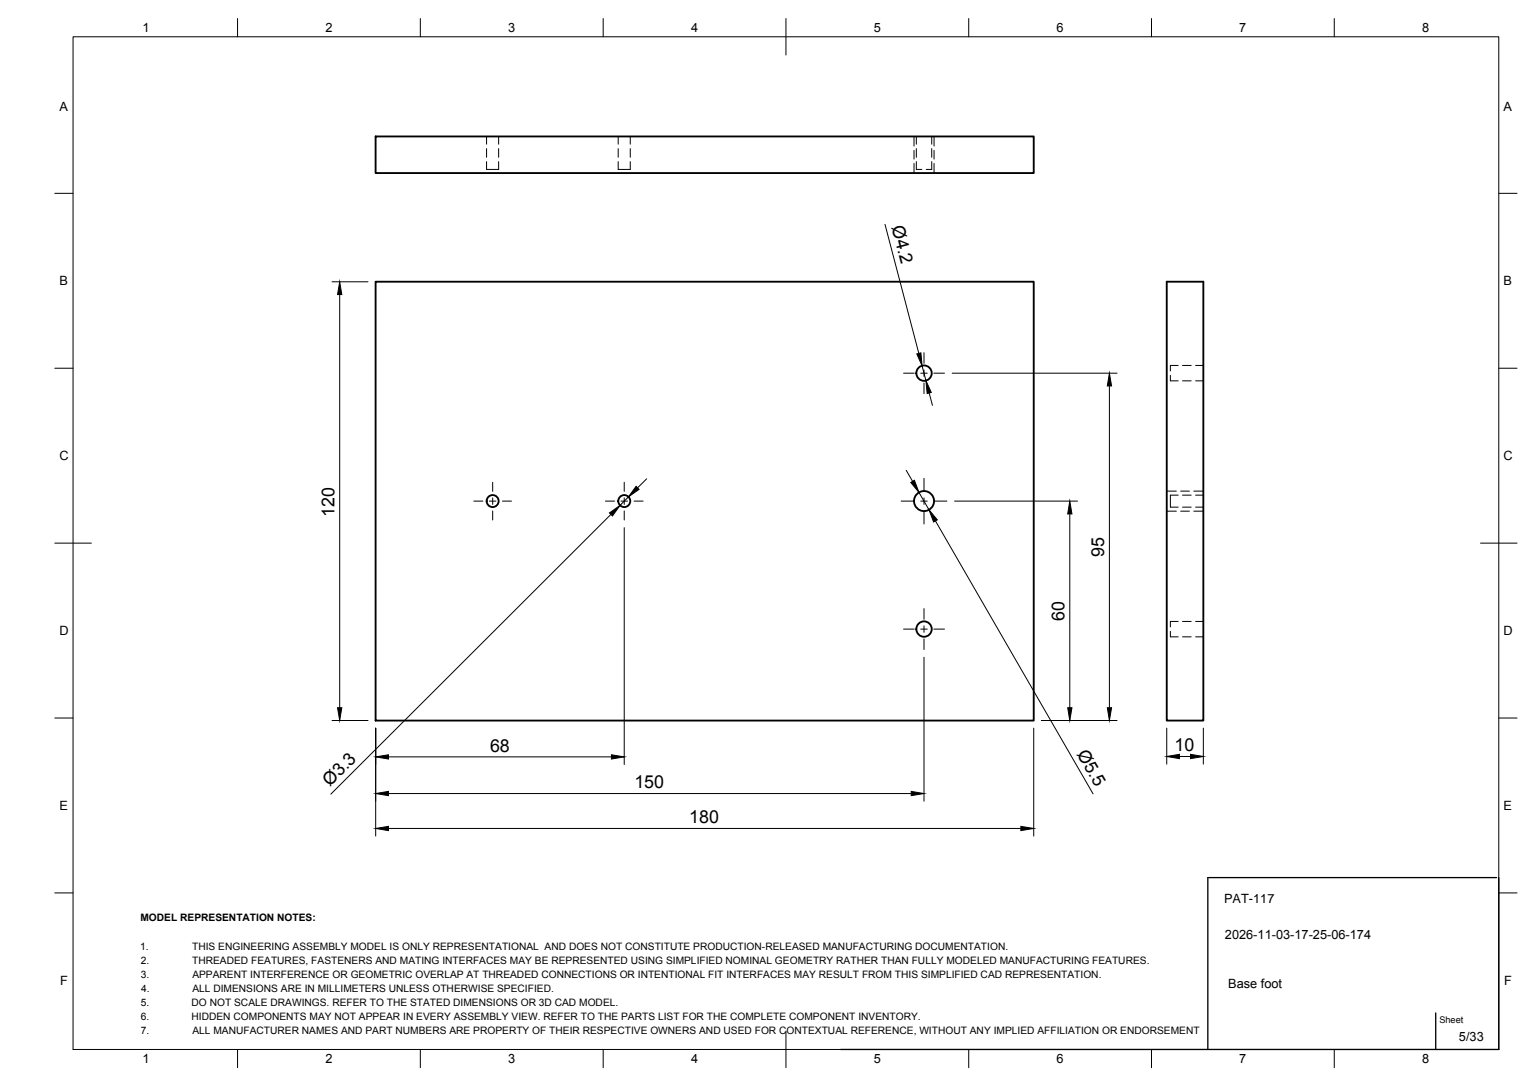
ISO-10303-21;
HEADER;
/* Generated by software containing ST-Developer
 * from STEP Tools, Inc. (www.steptools.com) 
 */

FILE_DESCRIPTION(
/* description */ ('Counterbalanced vertical column'),
/* implementation_level */ '2;1');

FILE_NAME(
/* name */ 'Base foot.step',
/* time_stamp */ '2026-10-29T16:47:22-07:00',
/* author */ (''),
/* organization */ (''),
/* preprocessor_version */ 'ST-DEVELOPER v20.2',
/* originating_system */ 'Autodesk Translation Framework v15.17.0.0',
/* authorisation */ '');

FILE_SCHEMA (('AUTOMOTIVE_DESIGN { 1 0 10303 214 3 1 1 }'));
ENDSEC;

DATA;
#10=MECHANICAL_DESIGN_GEOMETRIC_PRESENTATION_REPRESENTATION('',(#350),#15040);
#280=SHAPE_REPRESENTATION_RELATIONSHIP('SRR','None',#15184,#315);
#315=ADVANCED_BREP_SHAPE_REPRESENTATION('',(#385),#15003);
#350=STYLED_ITEM('',(#15436),#385);
#385=MANIFOLD_SOLID_BREP('Body1',#7073);
#416=FACE_BOUND('',#1245,.T.);
#417=FACE_BOUND('',#1246,.T.);
#418=FACE_BOUND('',#1247,.T.);
#419=FACE_BOUND('',#1248,.T.);
#420=FACE_BOUND('',#1249,.T.);
#421=FACE_BOUND('',#1251,.T.);
#531=PLANE('',#7504);
#532=PLANE('',#7508);
#533=PLANE('',#7512);
#534=PLANE('',#7516);
#535=PLANE('',#7520);
#536=PLANE('',#7521);
#537=PLANE('',#7522);
#538=PLANE('',#7523);
#539=PLANE('',#7524);
#540=PLANE('',#7525);
#826=FACE_OUTER_BOUND('',#1231,.T.);
#827=FACE_OUTER_BOUND('',#1232,.T.);
#828=FACE_OUTER_BOUND('',#1233,.T.);
#829=FACE_OUTER_BOUND('',#1234,.T.);
#830=FACE_OUTER_BOUND('',#1235,.T.);
#831=FACE_OUTER_BOUND('',#1236,.T.);
#832=FACE_OUTER_BOUND('',#1237,.T.);
#833=FACE_OUTER_BOUND('',#1238,.T.);
#834=FACE_OUTER_BOUND('',#1239,.T.);
#835=FACE_OUTER_BOUND('',#1240,.T.);
#836=FACE_OUTER_BOUND('',#1241,.T.);
#837=FACE_OUTER_BOUND('',#1242,.T.);
#838=FACE_OUTER_BOUND('',#1243,.T.);
#839=FACE_OUTER_BOUND('',#1244,.T.);
#840=FACE_OUTER_BOUND('',#1250,.T.);
#1231=EDGE_LOOP('',(#4788,#4789,#4790,#4791));
#1232=EDGE_LOOP('',(#4792));
#1233=EDGE_LOOP('',(#4793,#4794,#4795,#4796));
#1234=EDGE_LOOP('',(#4797));
#1235=EDGE_LOOP('',(#4798,#4799,#4800,#4801));
#1236=EDGE_LOOP('',(#4802));
#1237=EDGE_LOOP('',(#4803,#4804,#4805,#4806));
#1238=EDGE_LOOP('',(#4807));
#1239=EDGE_LOOP('',(#4808,#4809,#4810,#4811));
#1240=EDGE_LOOP('',(#4812,#4813,#4814,#4815));
#1241=EDGE_LOOP('',(#4816,#4817,#4818,#4819));
#1242=EDGE_LOOP('',(#4820,#4821,#4822,#4823));
#1243=EDGE_LOOP('',(#4824,#4825,#4826,#4827));
#1244=EDGE_LOOP('',(#4828,#4829,#4830,#4831));
#1245=EDGE_LOOP('',(#4832));
#1246=EDGE_LOOP('',(#4833));
#1247=EDGE_LOOP('',(#4834));
#1248=EDGE_LOOP('',(#4835));
#1249=EDGE_LOOP('',(#4836));
#1250=EDGE_LOOP('',(#4837,#4838,#4839,#4840));
#1251=EDGE_LOOP('',(#4841));
#1751=LINE('',#10345,#2422);
#1752=LINE('',#10352,#2423);
#1753=LINE('',#10359,#2424);
#1754=LINE('',#10366,#2425);
#1755=LINE('',#10373,#2426);
#1756=LINE('',#10378,#2427);
#1757=LINE('',#10380,#2428);
#1758=LINE('',#10382,#2429);
#1759=LINE('',#10383,#2430);
#1760=LINE('',#10386,#2431);
#1761=LINE('',#10388,#2432);
#1762=LINE('',#10389,#2433);
#1763=LINE('',#10392,#2434);
#1764=LINE('',#10394,#2435);
#1765=LINE('',#10395,#2436);
#1766=LINE('',#10397,#2437);
#1767=LINE('',#10398,#2438);
#2422=VECTOR('',#8231,0.21);
#2423=VECTOR('',#8240,0.21);
#2424=VECTOR('',#8249,0.165);
#2425=VECTOR('',#8258,0.164999999999999);
#2426=VECTOR('',#8267,0.275);
#2427=VECTOR('',#8272,1.);
#2428=VECTOR('',#8273,1.);
#2429=VECTOR('',#8274,1.);
#2430=VECTOR('',#8275,1.);
#2431=VECTOR('',#8278,1.);
#2432=VECTOR('',#8279,1.);
#2433=VECTOR('',#8280,1.);
#2434=VECTOR('',#8283,1.);
#2435=VECTOR('',#8284,1.);
#2436=VECTOR('',#8285,1.);
#2437=VECTOR('',#8288,1.);
#2438=VECTOR('',#8289,1.);
#3093=CIRCLE('',#7502,0.21);
#3094=CIRCLE('',#7503,0.21);
#3095=CIRCLE('',#7506,0.21);
#3096=CIRCLE('',#7507,0.21);
#3097=CIRCLE('',#7510,0.165);
#3098=CIRCLE('',#7511,0.165);
#3099=CIRCLE('',#7514,0.164999999999999);
#3100=CIRCLE('',#7515,0.164999999999999);
#3101=CIRCLE('',#7518,0.275);
#3102=CIRCLE('',#7519,0.275);
#3306=VERTEX_POINT('',#10342);
#3307=VERTEX_POINT('',#10344);
#3308=VERTEX_POINT('',#10349);
#3309=VERTEX_POINT('',#10351);
#3310=VERTEX_POINT('',#10356);
#3311=VERTEX_POINT('',#10358);
#3312=VERTEX_POINT('',#10363);
#3313=VERTEX_POINT('',#10365);
#3314=VERTEX_POINT('',#10370);
#3315=VERTEX_POINT('',#10372);
#3316=VERTEX_POINT('',#10376);
#3317=VERTEX_POINT('',#10377);
#3318=VERTEX_POINT('',#10379);
#3319=VERTEX_POINT('',#10381);
#3320=VERTEX_POINT('',#10385);
#3321=VERTEX_POINT('',#10387);
#3322=VERTEX_POINT('',#10391);
#3323=VERTEX_POINT('',#10393);
#3895=EDGE_CURVE('',#3306,#3306,#3093,.T.);
#3896=EDGE_CURVE('',#3306,#3307,#1751,.T.);
#3897=EDGE_CURVE('',#3307,#3307,#3094,.T.);
#3898=EDGE_CURVE('',#3308,#3308,#3095,.T.);
#3899=EDGE_CURVE('',#3308,#3309,#1752,.T.);
#3900=EDGE_CURVE('',#3309,#3309,#3096,.T.);
#3901=EDGE_CURVE('',#3310,#3310,#3097,.T.);
#3902=EDGE_CURVE('',#3310,#3311,#1753,.T.);
#3903=EDGE_CURVE('',#3311,#3311,#3098,.T.);
#3904=EDGE_CURVE('',#3312,#3312,#3099,.T.);
#3905=EDGE_CURVE('',#3312,#3313,#1754,.T.);
#3906=EDGE_CURVE('',#3313,#3313,#3100,.T.);
#3907=EDGE_CURVE('',#3314,#3314,#3101,.T.);
#3908=EDGE_CURVE('',#3314,#3315,#1755,.T.);
#3909=EDGE_CURVE('',#3315,#3315,#3102,.T.);
#3910=EDGE_CURVE('',#3316,#3317,#1756,.T.);
#3911=EDGE_CURVE('',#3317,#3318,#1757,.T.);
#3912=EDGE_CURVE('',#3319,#3318,#1758,.T.);
#3913=EDGE_CURVE('',#3316,#3319,#1759,.T.);
#3914=EDGE_CURVE('',#3320,#3316,#1760,.T.);
#3915=EDGE_CURVE('',#3321,#3319,#1761,.T.);
#3916=EDGE_CURVE('',#3320,#3321,#1762,.T.);
#3917=EDGE_CURVE('',#3322,#3320,#1763,.T.);
#3918=EDGE_CURVE('',#3323,#3321,#1764,.T.);
#3919=EDGE_CURVE('',#3322,#3323,#1765,.T.);
#3920=EDGE_CURVE('',#3317,#3322,#1766,.T.);
#3921=EDGE_CURVE('',#3318,#3323,#1767,.T.);
#4788=ORIENTED_EDGE('',*,*,#3895,.F.);
#4789=ORIENTED_EDGE('',*,*,#3896,.T.);
#4790=ORIENTED_EDGE('',*,*,#3897,.F.);
#4791=ORIENTED_EDGE('',*,*,#3896,.F.);
#4792=ORIENTED_EDGE('',*,*,#3895,.T.);
#4793=ORIENTED_EDGE('',*,*,#3898,.F.);
#4794=ORIENTED_EDGE('',*,*,#3899,.T.);
#4795=ORIENTED_EDGE('',*,*,#3900,.F.);
#4796=ORIENTED_EDGE('',*,*,#3899,.F.);
#4797=ORIENTED_EDGE('',*,*,#3898,.T.);
#4798=ORIENTED_EDGE('',*,*,#3901,.F.);
#4799=ORIENTED_EDGE('',*,*,#3902,.T.);
#4800=ORIENTED_EDGE('',*,*,#3903,.F.);
#4801=ORIENTED_EDGE('',*,*,#3902,.F.);
#4802=ORIENTED_EDGE('',*,*,#3901,.T.);
#4803=ORIENTED_EDGE('',*,*,#3904,.F.);
#4804=ORIENTED_EDGE('',*,*,#3905,.T.);
#4805=ORIENTED_EDGE('',*,*,#3906,.F.);
#4806=ORIENTED_EDGE('',*,*,#3905,.F.);
#4807=ORIENTED_EDGE('',*,*,#3904,.T.);
#4808=ORIENTED_EDGE('',*,*,#3907,.F.);
#4809=ORIENTED_EDGE('',*,*,#3908,.T.);
#4810=ORIENTED_EDGE('',*,*,#3909,.F.);
#4811=ORIENTED_EDGE('',*,*,#3908,.F.);
#4812=ORIENTED_EDGE('',*,*,#3910,.T.);
#4813=ORIENTED_EDGE('',*,*,#3911,.T.);
#4814=ORIENTED_EDGE('',*,*,#3912,.F.);
#4815=ORIENTED_EDGE('',*,*,#3913,.F.);
#4816=ORIENTED_EDGE('',*,*,#3914,.T.);
#4817=ORIENTED_EDGE('',*,*,#3913,.T.);
#4818=ORIENTED_EDGE('',*,*,#3915,.F.);
#4819=ORIENTED_EDGE('',*,*,#3916,.F.);
#4820=ORIENTED_EDGE('',*,*,#3917,.T.);
#4821=ORIENTED_EDGE('',*,*,#3916,.T.);
#4822=ORIENTED_EDGE('',*,*,#3918,.F.);
#4823=ORIENTED_EDGE('',*,*,#3919,.F.);
#4824=ORIENTED_EDGE('',*,*,#3920,.T.);
#4825=ORIENTED_EDGE('',*,*,#3919,.T.);
#4826=ORIENTED_EDGE('',*,*,#3921,.F.);
#4827=ORIENTED_EDGE('',*,*,#3911,.F.);
#4828=ORIENTED_EDGE('',*,*,#3921,.T.);
#4829=ORIENTED_EDGE('',*,*,#3918,.T.);
#4830=ORIENTED_EDGE('',*,*,#3915,.T.);
#4831=ORIENTED_EDGE('',*,*,#3912,.T.);
#4832=ORIENTED_EDGE('',*,*,#3897,.T.);
#4833=ORIENTED_EDGE('',*,*,#3900,.T.);
#4834=ORIENTED_EDGE('',*,*,#3903,.T.);
#4835=ORIENTED_EDGE('',*,*,#3906,.T.);
#4836=ORIENTED_EDGE('',*,*,#3909,.T.);
#4837=ORIENTED_EDGE('',*,*,#3920,.F.);
#4838=ORIENTED_EDGE('',*,*,#3910,.F.);
#4839=ORIENTED_EDGE('',*,*,#3914,.F.);
#4840=ORIENTED_EDGE('',*,*,#3917,.F.);
#4841=ORIENTED_EDGE('',*,*,#3907,.T.);
#6574=CYLINDRICAL_SURFACE('',#7501,0.21);
#6575=CYLINDRICAL_SURFACE('',#7505,0.21);
#6576=CYLINDRICAL_SURFACE('',#7509,0.165);
#6577=CYLINDRICAL_SURFACE('',#7513,0.164999999999999);
#6578=CYLINDRICAL_SURFACE('',#7517,0.275);
#6668=ADVANCED_FACE('',(#826),#6574,.F.);
#6669=ADVANCED_FACE('',(#827),#531,.T.);
#6670=ADVANCED_FACE('',(#828),#6575,.F.);
#6671=ADVANCED_FACE('',(#829),#532,.T.);
#6672=ADVANCED_FACE('',(#830),#6576,.F.);
#6673=ADVANCED_FACE('',(#831),#533,.T.);
#6674=ADVANCED_FACE('',(#832),#6577,.F.);
#6675=ADVANCED_FACE('',(#833),#534,.T.);
#6676=ADVANCED_FACE('',(#834),#6578,.F.);
#6677=ADVANCED_FACE('',(#835),#535,.T.);
#6678=ADVANCED_FACE('',(#836),#536,.T.);
#6679=ADVANCED_FACE('',(#837),#537,.T.);
#6680=ADVANCED_FACE('',(#838),#538,.T.);
#6681=ADVANCED_FACE('',(#839,#416,#417,#418,#419,#420),#539,.T.);
#6682=ADVANCED_FACE('',(#840,#421),#540,.F.);
#7073=CLOSED_SHELL('',(#6668,#6669,#6670,#6671,#6672,#6673,#6674,#6675,
#6676,#6677,#6678,#6679,#6680,#6681,#6682));
#7500=AXIS2_PLACEMENT_3D('',#10340,#8225,#8226);
#7501=AXIS2_PLACEMENT_3D('',#10341,#8227,#8228);
#7502=AXIS2_PLACEMENT_3D('',#10343,#8229,#8230);
#7503=AXIS2_PLACEMENT_3D('',#10346,#8232,#8233);
#7504=AXIS2_PLACEMENT_3D('',#10347,#8234,#8235);
#7505=AXIS2_PLACEMENT_3D('',#10348,#8236,#8237);
#7506=AXIS2_PLACEMENT_3D('',#10350,#8238,#8239);
#7507=AXIS2_PLACEMENT_3D('',#10353,#8241,#8242);
#7508=AXIS2_PLACEMENT_3D('',#10354,#8243,#8244);
#7509=AXIS2_PLACEMENT_3D('',#10355,#8245,#8246);
#7510=AXIS2_PLACEMENT_3D('',#10357,#8247,#8248);
#7511=AXIS2_PLACEMENT_3D('',#10360,#8250,#8251);
#7512=AXIS2_PLACEMENT_3D('',#10361,#8252,#8253);
#7513=AXIS2_PLACEMENT_3D('',#10362,#8254,#8255);
#7514=AXIS2_PLACEMENT_3D('',#10364,#8256,#8257);
#7515=AXIS2_PLACEMENT_3D('',#10367,#8259,#8260);
#7516=AXIS2_PLACEMENT_3D('',#10368,#8261,#8262);
#7517=AXIS2_PLACEMENT_3D('',#10369,#8263,#8264);
#7518=AXIS2_PLACEMENT_3D('',#10371,#8265,#8266);
#7519=AXIS2_PLACEMENT_3D('',#10374,#8268,#8269);
#7520=AXIS2_PLACEMENT_3D('',#10375,#8270,#8271);
#7521=AXIS2_PLACEMENT_3D('',#10384,#8276,#8277);
#7522=AXIS2_PLACEMENT_3D('',#10390,#8281,#8282);
#7523=AXIS2_PLACEMENT_3D('',#10396,#8286,#8287);
#7524=AXIS2_PLACEMENT_3D('',#10399,#8290,#8291);
#7525=AXIS2_PLACEMENT_3D('',#10400,#8292,#8293);
#8225=DIRECTION('axis',(0.,0.,1.));
#8226=DIRECTION('refdir',(1.,0.,0.));
#8227=DIRECTION('center_axis',(0.,0.,1.));
#8228=DIRECTION('ref_axis',(1.,0.,0.));
#8229=DIRECTION('center_axis',(0.,0.,1.));
#8230=DIRECTION('ref_axis',(1.,0.,0.));
#8231=DIRECTION('',(0.,0.,1.));
#8232=DIRECTION('center_axis',(0.,0.,-1.));
#8233=DIRECTION('ref_axis',(1.,0.,0.));
#8234=DIRECTION('center_axis',(0.,0.,1.));
#8235=DIRECTION('ref_axis',(1.,0.,0.));
#8236=DIRECTION('center_axis',(0.,0.,1.));
#8237=DIRECTION('ref_axis',(1.,0.,0.));
#8238=DIRECTION('center_axis',(0.,0.,1.));
#8239=DIRECTION('ref_axis',(1.,0.,0.));
#8240=DIRECTION('',(0.,0.,1.));
#8241=DIRECTION('center_axis',(0.,0.,-1.));
#8242=DIRECTION('ref_axis',(1.,0.,0.));
#8243=DIRECTION('center_axis',(0.,0.,1.));
#8244=DIRECTION('ref_axis',(1.,0.,0.));
#8245=DIRECTION('center_axis',(0.,0.,1.));
#8246=DIRECTION('ref_axis',(1.,0.,0.));
#8247=DIRECTION('center_axis',(0.,0.,1.));
#8248=DIRECTION('ref_axis',(1.,0.,0.));
#8249=DIRECTION('',(0.,0.,1.));
#8250=DIRECTION('center_axis',(0.,0.,-1.));
#8251=DIRECTION('ref_axis',(1.,0.,0.));
#8252=DIRECTION('center_axis',(0.,0.,1.));
#8253=DIRECTION('ref_axis',(1.,0.,0.));
#8254=DIRECTION('center_axis',(0.,0.,1.));
#8255=DIRECTION('ref_axis',(1.,0.,0.));
#8256=DIRECTION('center_axis',(0.,0.,1.));
#8257=DIRECTION('ref_axis',(1.,0.,0.));
#8258=DIRECTION('',(0.,0.,1.));
#8259=DIRECTION('center_axis',(0.,0.,-1.));
#8260=DIRECTION('ref_axis',(1.,0.,0.));
#8261=DIRECTION('center_axis',(0.,0.,1.));
#8262=DIRECTION('ref_axis',(1.,0.,0.));
#8263=DIRECTION('center_axis',(0.,0.,1.));
#8264=DIRECTION('ref_axis',(1.,0.,0.));
#8265=DIRECTION('center_axis',(0.,0.,1.));
#8266=DIRECTION('ref_axis',(1.,0.,0.));
#8267=DIRECTION('',(0.,0.,1.));
#8268=DIRECTION('center_axis',(0.,0.,-1.));
#8269=DIRECTION('ref_axis',(1.,0.,0.));
#8270=DIRECTION('center_axis',(0.,1.,0.));
#8271=DIRECTION('ref_axis',(-1.,0.,0.));
#8272=DIRECTION('',(-1.,0.,0.));
#8273=DIRECTION('',(0.,0.,1.));
#8274=DIRECTION('',(-1.,0.,0.));
#8275=DIRECTION('',(0.,0.,1.));
#8276=DIRECTION('center_axis',(1.,0.,0.));
#8277=DIRECTION('ref_axis',(0.,1.,0.));
#8278=DIRECTION('',(0.,1.,0.));
#8279=DIRECTION('',(0.,1.,0.));
#8280=DIRECTION('',(0.,0.,1.));
#8281=DIRECTION('center_axis',(0.,-1.,0.));
#8282=DIRECTION('ref_axis',(1.,0.,0.));
#8283=DIRECTION('',(1.,0.,0.));
#8284=DIRECTION('',(1.,0.,0.));
#8285=DIRECTION('',(0.,0.,1.));
#8286=DIRECTION('center_axis',(-1.,0.,0.));
#8287=DIRECTION('ref_axis',(0.,-1.,0.));
#8288=DIRECTION('',(0.,-1.,0.));
#8289=DIRECTION('',(0.,-1.,0.));
#8290=DIRECTION('center_axis',(0.,0.,1.));
#8291=DIRECTION('ref_axis',(1.,0.,0.));
#8292=DIRECTION('center_axis',(0.,0.,1.));
#8293=DIRECTION('ref_axis',(1.,0.,0.));
#10340=CARTESIAN_POINT('',(0.,0.,0.));
#10341=CARTESIAN_POINT('Origin',(3.,3.5,-0.9));
#10342=CARTESIAN_POINT('',(2.79,3.5,-0.9));
#10343=CARTESIAN_POINT('Origin',(3.,3.5,-0.9));
#10344=CARTESIAN_POINT('',(2.79,3.5,0.));
#10345=CARTESIAN_POINT('',(2.79,3.5,-0.9));
#10346=CARTESIAN_POINT('Origin',(3.,3.5,0.));
#10347=CARTESIAN_POINT('Origin',(3.,3.5,-0.9));
#10348=CARTESIAN_POINT('Origin',(3.,-3.5,-0.9));
#10349=CARTESIAN_POINT('',(2.79,-3.5,-0.9));
#10350=CARTESIAN_POINT('Origin',(3.,-3.5,-0.9));
#10351=CARTESIAN_POINT('',(2.79,-3.5,0.));
#10352=CARTESIAN_POINT('',(2.79,-3.5,-0.9));
#10353=CARTESIAN_POINT('Origin',(3.,-3.5,0.));
#10354=CARTESIAN_POINT('Origin',(3.,-3.5,-0.9));
#10355=CARTESIAN_POINT('Origin',(-5.2,0.,-0.9));
#10356=CARTESIAN_POINT('',(-5.365,-2.02066721859313E-17,-0.9));
#10357=CARTESIAN_POINT('Origin',(-5.2,0.,-0.9));
#10358=CARTESIAN_POINT('',(-5.365,2.02066721859313E-17,0.));
#10359=CARTESIAN_POINT('',(-5.365,-2.02066721859313E-17,-0.9));
#10360=CARTESIAN_POINT('Origin',(-5.2,0.,0.));
#10361=CARTESIAN_POINT('Origin',(-5.2,0.,-0.9));
#10362=CARTESIAN_POINT('Origin',(-8.8,0.,-0.9));
#10363=CARTESIAN_POINT('',(-8.965,-2.02066721859312E-17,-0.9));
#10364=CARTESIAN_POINT('Origin',(-8.8,0.,-0.9));
#10365=CARTESIAN_POINT('',(-8.965,2.02066721859312E-17,0.));
#10366=CARTESIAN_POINT('',(-8.965,-2.02066721859312E-17,-0.9));
#10367=CARTESIAN_POINT('Origin',(-8.8,0.,0.));
#10368=CARTESIAN_POINT('Origin',(-8.8,0.,-0.9));
#10369=CARTESIAN_POINT('Origin',(3.,0.,-1.1));
#10370=CARTESIAN_POINT('',(2.725,-3.36777869765522E-17,-1.));
#10371=CARTESIAN_POINT('Origin',(3.,0.,-1.));
#10372=CARTESIAN_POINT('',(2.725,3.36777869765522E-17,0.));
#10373=CARTESIAN_POINT('',(2.725,-3.36777869765522E-17,-1.1));
#10374=CARTESIAN_POINT('Origin',(3.,0.,0.));
#10375=CARTESIAN_POINT('Origin',(6.,6.,-1.));
#10376=CARTESIAN_POINT('',(6.,6.,-1.));
#10377=CARTESIAN_POINT('',(-12.,6.,-1.));
#10378=CARTESIAN_POINT('',(6.,6.,-1.));
#10379=CARTESIAN_POINT('',(-12.,6.,0.));
#10380=CARTESIAN_POINT('',(-12.,6.,-1.));
#10381=CARTESIAN_POINT('',(6.,6.,0.));
#10382=CARTESIAN_POINT('',(6.,6.,0.));
#10383=CARTESIAN_POINT('',(6.,6.,-1.));
#10384=CARTESIAN_POINT('Origin',(6.,-6.,-1.));
#10385=CARTESIAN_POINT('',(6.,-6.,-1.));
#10386=CARTESIAN_POINT('',(6.,-6.,-1.));
#10387=CARTESIAN_POINT('',(6.,-6.,0.));
#10388=CARTESIAN_POINT('',(6.,-6.,0.));
#10389=CARTESIAN_POINT('',(6.,-6.,-1.));
#10390=CARTESIAN_POINT('Origin',(-12.,-6.,-1.));
#10391=CARTESIAN_POINT('',(-12.,-6.,-1.));
#10392=CARTESIAN_POINT('',(-12.,-6.,-1.));
#10393=CARTESIAN_POINT('',(-12.,-6.,0.));
#10394=CARTESIAN_POINT('',(-12.,-6.,0.));
#10395=CARTESIAN_POINT('',(-12.,-6.,-1.));
#10396=CARTESIAN_POINT('Origin',(-12.,6.,-1.));
#10397=CARTESIAN_POINT('',(-12.,6.,-1.));
#10398=CARTESIAN_POINT('',(-12.,6.,0.));
#10399=CARTESIAN_POINT('Origin',(-3.,0.,0.));
#10400=CARTESIAN_POINT('Origin',(-3.,0.,-1.));
#14963=UNCERTAINTY_MEASURE_WITH_UNIT(LENGTH_MEASURE(0.001),#15041,
'DISTANCE_ACCURACY_VALUE',
'Maximum model space distance between geometric entities at asserted c
onnectivities');
#15000=UNCERTAINTY_MEASURE_WITH_UNIT(LENGTH_MEASURE(0.001),#15041,
'DISTANCE_ACCURACY_VALUE',
'Maximum model space distance between geometric entities at asserted c
onnectivities');
#15003=(
GEOMETRIC_REPRESENTATION_CONTEXT(3)
GLOBAL_UNCERTAINTY_ASSIGNED_CONTEXT((#14963))
GLOBAL_UNIT_ASSIGNED_CONTEXT((#15041,#15043,#15044))
REPRESENTATION_CONTEXT('','3D')
);
#15040=(
GEOMETRIC_REPRESENTATION_CONTEXT(3)
GLOBAL_UNCERTAINTY_ASSIGNED_CONTEXT((#15000))
GLOBAL_UNIT_ASSIGNED_CONTEXT((#15041,#15043,#15044))
REPRESENTATION_CONTEXT('','3D')
);
#15041=(
LENGTH_UNIT()
NAMED_UNIT(*)
SI_UNIT(.CENTI.,.METRE.)
);
#15043=(
NAMED_UNIT(*)
PLANE_ANGLE_UNIT()
SI_UNIT($,.RADIAN.)
);
#15044=(
NAMED_UNIT(*)
SI_UNIT($,.STERADIAN.)
SOLID_ANGLE_UNIT()
);
#15047=SHAPE_DEFINITION_REPRESENTATION(#15086,#15184);
#15086=PRODUCT_DEFINITION_SHAPE('',$,#15224);
#15184=SHAPE_REPRESENTATION('',(#7500),#15003);
#15221=PRODUCT_DEFINITION_CONTEXT('part definition',#15340,'design');
#15224=PRODUCT_DEFINITION('Base foot','Base foot',#15263,#15221);
#15263=PRODUCT_DEFINITION_FORMATION('',$,#15344);
#15340=APPLICATION_CONTEXT(
'Core Data for Automotive Mechanical Design Process');
#15341=PRODUCT_CONTEXT('part definition',#15340,'mechanical');
#15344=PRODUCT('Base foot','Base foot','Base foot',(#15341));
#15430=COLOUR_RGB('Dark Blue',0.08,0.2,0.34);
#15431=FILL_AREA_STYLE_COLOUR('',#15430);
#15432=FILL_AREA_STYLE('',(#15431));
#15433=SURFACE_STYLE_FILL_AREA(#15432);
#15434=SURFACE_SIDE_STYLE('',(#15433));
#15435=SURFACE_STYLE_USAGE(.BOTH.,#15434);
#15436=PRESENTATION_STYLE_ASSIGNMENT((#15435));
ENDSEC;
END-ISO-10303-21;
